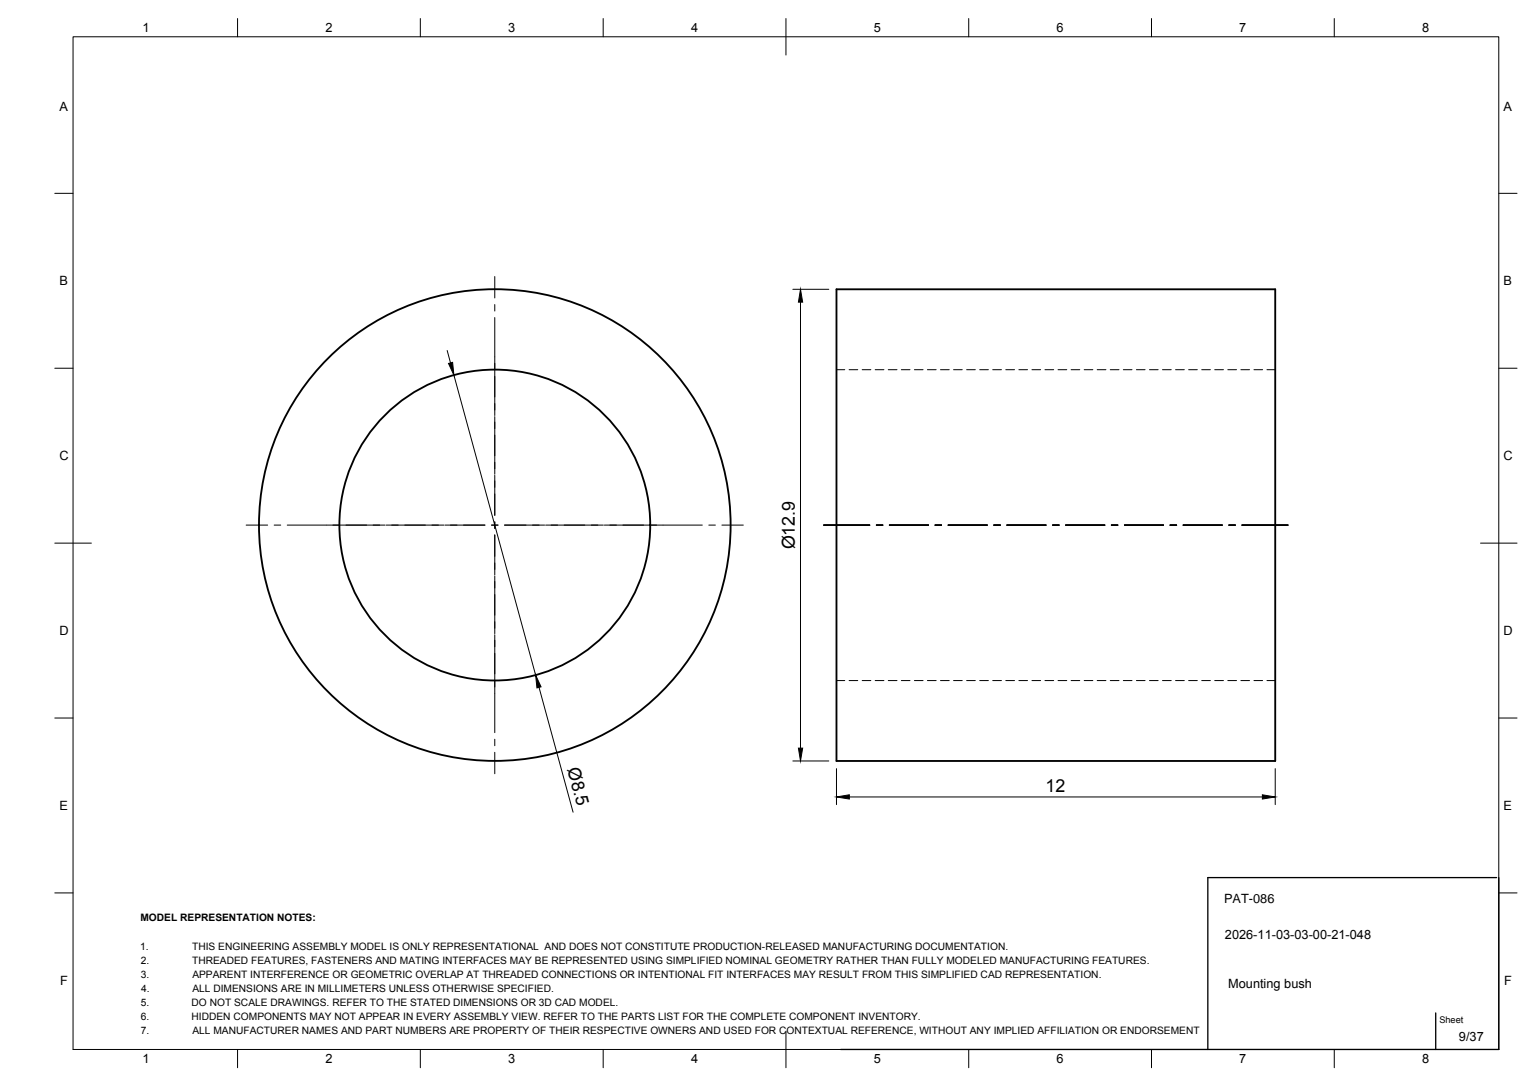
ISO-10303-21;
HEADER;
/* Generated by software containing ST-Developer
 * from STEP Tools, Inc. (www.steptools.com) 
 */

FILE_DESCRIPTION(
/* description */ ('Ratchet and pawl hand winch drum'),
/* implementation_level */ '2;1');

FILE_NAME(
/* name */ 'Mounting bush.step',
/* time_stamp */ '2026-10-27T12:42:58-07:00',
/* author */ (''),
/* organization */ (''),
/* preprocessor_version */ 'ST-DEVELOPER v20.2',
/* originating_system */ 'Autodesk Translation Framework v15.17.0.0',
/* authorisation */ '');

FILE_SCHEMA (('AUTOMOTIVE_DESIGN { 1 0 10303 214 3 1 1 }'));
ENDSEC;

DATA;
#10=MECHANICAL_DESIGN_GEOMETRIC_PRESENTATION_REPRESENTATION('',(#393),#11801);
#325=SHAPE_REPRESENTATION_RELATIONSHIP('SRR','None',#11951,#359);
#359=ADVANCED_BREP_SHAPE_REPRESENTATION('',(#428),#11768);
#393=STYLED_ITEM('',(#12206),#428);
#428=MANIFOLD_SOLID_BREP('Body1',#6270);
#492=FACE_BOUND('',#1283,.T.);
#493=FACE_BOUND('',#1285,.T.);
#629=PLANE('',#6780);
#630=PLANE('',#6781);
#888=FACE_OUTER_BOUND('',#1280,.T.);
#889=FACE_OUTER_BOUND('',#1281,.T.);
#890=FACE_OUTER_BOUND('',#1282,.T.);
#891=FACE_OUTER_BOUND('',#1284,.T.);
#1280=EDGE_LOOP('',(#4463,#4464,#4465,#4466));
#1281=EDGE_LOOP('',(#4467,#4468,#4469,#4470));
#1282=EDGE_LOOP('',(#4471));
#1283=EDGE_LOOP('',(#4472));
#1284=EDGE_LOOP('',(#4473));
#1285=EDGE_LOOP('',(#4474));
#1765=LINE('',#9466,#2276);
#1766=LINE('',#9472,#2277);
#2276=VECTOR('',#7620,0.425);
#2277=VECTOR('',#7627,0.645);
#2759=CIRCLE('',#6775,0.425);
#2760=CIRCLE('',#6776,0.425);
#2761=CIRCLE('',#6778,0.645);
#2762=CIRCLE('',#6779,0.645);
#3014=VERTEX_POINT('',#9463);
#3015=VERTEX_POINT('',#9465);
#3016=VERTEX_POINT('',#9469);
#3017=VERTEX_POINT('',#9471);
#3575=EDGE_CURVE('',#3014,#3014,#2759,.T.);
#3576=EDGE_CURVE('',#3014,#3015,#1765,.T.);
#3577=EDGE_CURVE('',#3015,#3015,#2760,.T.);
#3578=EDGE_CURVE('',#3016,#3016,#2761,.T.);
#3579=EDGE_CURVE('',#3016,#3017,#1766,.T.);
#3580=EDGE_CURVE('',#3017,#3017,#2762,.T.);
#4463=ORIENTED_EDGE('',*,*,#3575,.F.);
#4464=ORIENTED_EDGE('',*,*,#3576,.T.);
#4465=ORIENTED_EDGE('',*,*,#3577,.T.);
#4466=ORIENTED_EDGE('',*,*,#3576,.F.);
#4467=ORIENTED_EDGE('',*,*,#3578,.F.);
#4468=ORIENTED_EDGE('',*,*,#3579,.T.);
#4469=ORIENTED_EDGE('',*,*,#3580,.T.);
#4470=ORIENTED_EDGE('',*,*,#3579,.F.);
#4471=ORIENTED_EDGE('',*,*,#3578,.T.);
#4472=ORIENTED_EDGE('',*,*,#3575,.T.);
#4473=ORIENTED_EDGE('',*,*,#3580,.F.);
#4474=ORIENTED_EDGE('',*,*,#3577,.F.);
#5827=CYLINDRICAL_SURFACE('',#6774,0.425);
#5828=CYLINDRICAL_SURFACE('',#6777,0.645);
#5958=ADVANCED_FACE('',(#888),#5827,.F.);
#5959=ADVANCED_FACE('',(#889),#5828,.T.);
#5960=ADVANCED_FACE('',(#890,#492),#629,.T.);
#5961=ADVANCED_FACE('',(#891,#493),#630,.F.);
#6270=CLOSED_SHELL('',(#5958,#5959,#5960,#5961));
#6773=AXIS2_PLACEMENT_3D('',#9461,#7614,#7615);
#6774=AXIS2_PLACEMENT_3D('',#9462,#7616,#7617);
#6775=AXIS2_PLACEMENT_3D('',#9464,#7618,#7619);
#6776=AXIS2_PLACEMENT_3D('',#9467,#7621,#7622);
#6777=AXIS2_PLACEMENT_3D('',#9468,#7623,#7624);
#6778=AXIS2_PLACEMENT_3D('',#9470,#7625,#7626);
#6779=AXIS2_PLACEMENT_3D('',#9473,#7628,#7629);
#6780=AXIS2_PLACEMENT_3D('',#9474,#7630,#7631);
#6781=AXIS2_PLACEMENT_3D('',#9475,#7632,#7633);
#7614=DIRECTION('axis',(0.,0.,1.));
#7615=DIRECTION('refdir',(1.,0.,0.));
#7616=DIRECTION('center_axis',(0.,0.,1.));
#7617=DIRECTION('ref_axis',(1.,0.,0.));
#7618=DIRECTION('center_axis',(0.,0.,-1.));
#7619=DIRECTION('ref_axis',(1.,0.,0.));
#7620=DIRECTION('',(0.,0.,-1.));
#7621=DIRECTION('center_axis',(0.,0.,-1.));
#7622=DIRECTION('ref_axis',(1.,0.,0.));
#7623=DIRECTION('center_axis',(0.,0.,1.));
#7624=DIRECTION('ref_axis',(1.,0.,0.));
#7625=DIRECTION('center_axis',(0.,0.,1.));
#7626=DIRECTION('ref_axis',(1.,0.,0.));
#7627=DIRECTION('',(0.,0.,-1.));
#7628=DIRECTION('center_axis',(0.,0.,1.));
#7629=DIRECTION('ref_axis',(1.,0.,0.));
#7630=DIRECTION('center_axis',(0.,0.,1.));
#7631=DIRECTION('ref_axis',(1.,0.,0.));
#7632=DIRECTION('center_axis',(0.,0.,1.));
#7633=DIRECTION('ref_axis',(1.,0.,0.));
#9461=CARTESIAN_POINT('',(0.,0.,0.));
#9462=CARTESIAN_POINT('Origin',(-4.75,0.,3.2));
#9463=CARTESIAN_POINT('',(-5.175,-5.20474889637625E-17,4.4));
#9464=CARTESIAN_POINT('Origin',(-4.75,0.,4.4));
#9465=CARTESIAN_POINT('',(-5.175,-5.20474889637625E-17,3.2));
#9466=CARTESIAN_POINT('',(-5.175,-5.20474889637625E-17,3.2));
#9467=CARTESIAN_POINT('Origin',(-4.75,0.,3.2));
#9468=CARTESIAN_POINT('Origin',(-4.75,0.,3.2));
#9469=CARTESIAN_POINT('',(-5.395,-7.89897185450042E-17,4.4));
#9470=CARTESIAN_POINT('Origin',(-4.75,0.,4.4));
#9471=CARTESIAN_POINT('',(-5.395,-7.89897185450042E-17,3.2));
#9472=CARTESIAN_POINT('',(-5.395,-7.89897185450042E-17,3.2));
#9473=CARTESIAN_POINT('Origin',(-4.75,0.,3.2));
#9474=CARTESIAN_POINT('Origin',(-4.75,0.,4.4));
#9475=CARTESIAN_POINT('Origin',(-4.75,0.,3.2));
#11728=UNCERTAINTY_MEASURE_WITH_UNIT(LENGTH_MEASURE(0.001),#11802,
'DISTANCE_ACCURACY_VALUE',
'Maximum model space distance between geometric entities at asserted c
onnectivities');
#11761=UNCERTAINTY_MEASURE_WITH_UNIT(LENGTH_MEASURE(0.001),#11802,
'DISTANCE_ACCURACY_VALUE',
'Maximum model space distance between geometric entities at asserted c
onnectivities');
#11768=(
GEOMETRIC_REPRESENTATION_CONTEXT(3)
GLOBAL_UNCERTAINTY_ASSIGNED_CONTEXT((#11728))
GLOBAL_UNIT_ASSIGNED_CONTEXT((#11802,#11804,#11805))
REPRESENTATION_CONTEXT('','3D')
);
#11801=(
GEOMETRIC_REPRESENTATION_CONTEXT(3)
GLOBAL_UNCERTAINTY_ASSIGNED_CONTEXT((#11761))
GLOBAL_UNIT_ASSIGNED_CONTEXT((#11802,#11804,#11805))
REPRESENTATION_CONTEXT('','3D')
);
#11802=(
LENGTH_UNIT()
NAMED_UNIT(*)
SI_UNIT(.CENTI.,.METRE.)
);
#11804=(
NAMED_UNIT(*)
PLANE_ANGLE_UNIT()
SI_UNIT($,.RADIAN.)
);
#11805=(
NAMED_UNIT(*)
SI_UNIT($,.STERADIAN.)
SOLID_ANGLE_UNIT()
);
#11812=SHAPE_DEFINITION_REPRESENTATION(#11851,#11951);
#11851=PRODUCT_DEFINITION_SHAPE('',$,#11991);
#11951=SHAPE_REPRESENTATION('',(#6773),#11768);
#11984=PRODUCT_DEFINITION_CONTEXT('part definition',#12103,'design');
#11991=PRODUCT_DEFINITION('Mounting bush','Mounting bush',#12030,#11984);
#12030=PRODUCT_DEFINITION_FORMATION('',$,#12111);
#12103=APPLICATION_CONTEXT(
'Core Data for Automotive Mechanical Design Process');
#12104=PRODUCT_CONTEXT('part definition',#12103,'mechanical');
#12111=PRODUCT('Mounting bush','Mounting bush','Mounting bush',(#12104));
#12200=COLOUR_RGB('Sky Blue',0.24,0.69,0.87);
#12201=FILL_AREA_STYLE_COLOUR('',#12200);
#12202=FILL_AREA_STYLE('',(#12201));
#12203=SURFACE_STYLE_FILL_AREA(#12202);
#12204=SURFACE_SIDE_STYLE('',(#12203));
#12205=SURFACE_STYLE_USAGE(.BOTH.,#12204);
#12206=PRESENTATION_STYLE_ASSIGNMENT((#12205));
ENDSEC;
END-ISO-10303-21;
